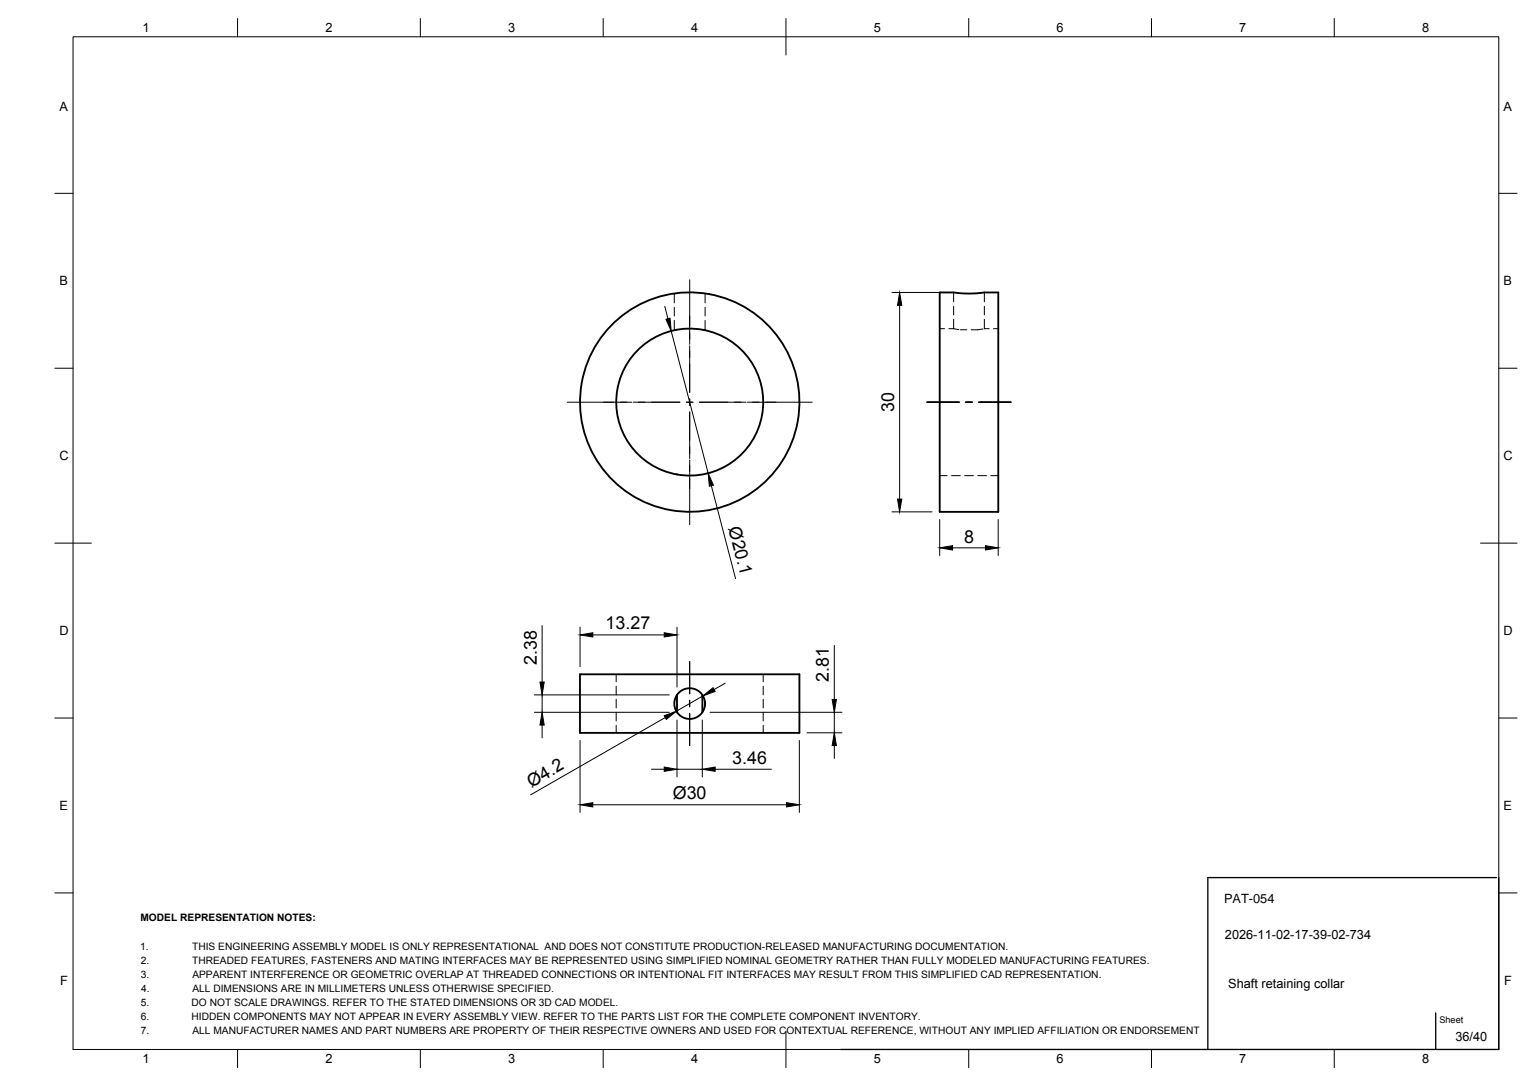
ISO-10303-21;
HEADER;
/* Generated by software containing ST-Developer
 * from STEP Tools, Inc. (www.steptools.com) 
 */

FILE_DESCRIPTION(
/* description */ ('PAT-054'),
/* implementation_level */ '2;1');

FILE_NAME(
/* name */ 'Shaft retaining collar.step',
/* time_stamp */ '2026-10-29T16:38:13-07:00',
/* author */ (''),
/* organization */ (''),
/* preprocessor_version */ 'ST-DEVELOPER v20.2',
/* originating_system */ 'Autodesk Translation Framework v15.17.0.0',
/* authorisation */ '');

FILE_SCHEMA (('AUTOMOTIVE_DESIGN { 1 0 10303 214 3 1 1 }'));
ENDSEC;

DATA;
#10=MECHANICAL_DESIGN_GEOMETRIC_PRESENTATION_REPRESENTATION('',(#950),#33981);
#737=B_SPLINE_CURVE_WITH_KNOTS('',3,(#33386,#33387,#33388,#33389,#33390,
#33391,#33392,#33393),.UNSPECIFIED.,.F.,.F.,(4,2,2,4),(0.756005737987019,
0.793568827564653,0.872922520054208,0.952276212543762),.UNSPECIFIED.);
#738=B_SPLINE_CURVE_WITH_KNOTS('',3,(#33396,#33397,#33398,#33399,#33400,
#33401,#33402,#33403,#33404,#33405,#33406,#33407,#33408,#33409),
 .UNSPECIFIED.,.F.,.F.,(4,2,2,2,2,2,4),(0.121154929624509,0.158718019202145,
0.238071711691699,0.317425404181254,0.396779096670809,0.476132789160363,
0.513695878738001),.UNSPECIFIED.);
#739=B_SPLINE_CURVE_WITH_KNOTS('',3,(#33410,#33411,#33412,#33413,#33414,
#33415,#33416,#33417),.UNSPECIFIED.,.F.,.F.,(4,2,2,4),(0.952276212543762,
1.03162990503332,1.11098359752287,1.14854668710052),.UNSPECIFIED.);
#740=B_SPLINE_CURVE_WITH_KNOTS('',3,(#33421,#33422,#33423,#33424,#33425,
#33426,#33427,#33428,#33429,#33430),.UNSPECIFIED.,.F.,.F.,(4,2,2,2,4),(0.,
0.0792165807733642,0.158433161546728,0.237648697074572,0.316864232602417),
 .UNSPECIFIED.);
#741=B_SPLINE_CURVE_WITH_KNOTS('',3,(#33431,#33432,#33433,#33434,#33435,
#33436,#33437,#33438,#33439,#33440,#33441,#33442,#33443,#33444,#33445,#33446,
#33447,#33448,#33449,#33450,#33451,#33452,#33453,#33454,#33455,#33456),
 .UNSPECIFIED.,.F.,.F.,(4,2,2,2,2,2,2,2,2,2,2,2,4),(0.316864232602417,0.396079768130261,
0.475295303658105,0.554511884431469,0.633728465204833,0.712945045978197,
0.792161626751562,0.871377162279406,0.95059269780725,1.02980823333509,1.10902376886294,
1.1882403496363,1.26745693040967),.UNSPECIFIED.);
#847=SHAPE_REPRESENTATION_RELATIONSHIP('SRR','None',#34225,#891);
#891=ADVANCED_BREP_SHAPE_REPRESENTATION('',(#1005),#33973);
#950=STYLED_ITEM('',(#34517),#1005);
#1005=MANIFOLD_SOLID_BREP('Body1',#13065);
#1210=FACE_BOUND('',#3152,.T.);
#1211=FACE_BOUND('',#3154,.T.);
#1212=FACE_BOUND('',#3156,.T.);
#1213=FACE_BOUND('',#3158,.T.);
#1527=PLANE('',#14711);
#1528=PLANE('',#14715);
#1529=PLANE('',#14722);
#1530=PLANE('',#14723);
#2227=FACE_OUTER_BOUND('',#3148,.T.);
#2228=FACE_OUTER_BOUND('',#3149,.T.);
#2229=FACE_OUTER_BOUND('',#3150,.T.);
#2230=FACE_OUTER_BOUND('',#3151,.T.);
#2231=FACE_OUTER_BOUND('',#3153,.T.);
#2232=FACE_OUTER_BOUND('',#3155,.T.);
#2233=FACE_OUTER_BOUND('',#3157,.T.);
#3148=EDGE_LOOP('',(#11681,#11682));
#3149=EDGE_LOOP('',(#11683,#11684,#11685,#11686,#11687,#11688,#11689,#11690,
#11691));
#3150=EDGE_LOOP('',(#11692,#11693));
#3151=EDGE_LOOP('',(#11694,#11695,#11696,#11697));
#3152=EDGE_LOOP('',(#11698,#11699,#11700,#11701,#11702));
#3153=EDGE_LOOP('',(#11703,#11704,#11705,#11706));
#3154=EDGE_LOOP('',(#11707,#11708));
#3155=EDGE_LOOP('',(#11709));
#3156=EDGE_LOOP('',(#11710));
#3157=EDGE_LOOP('',(#11711));
#3158=EDGE_LOOP('',(#11712));
#4072=LINE('',#33381,#5006);
#4073=LINE('',#33419,#5007);
#4074=LINE('',#33458,#5008);
#4075=LINE('',#33463,#5009);
#4076=LINE('',#33469,#5010);
#5006=VECTOR('',#18031,1.);
#5007=VECTOR('',#18038,0.210000000000001);
#5008=VECTOR('',#18041,1.);
#5009=VECTOR('',#18046,1.005);
#5010=VECTOR('',#18053,1.5);
#5530=CIRCLE('',#14712,0.210000000000001);
#5531=CIRCLE('',#14714,0.210000000000001);
#5532=CIRCLE('',#14717,1.005);
#5533=CIRCLE('',#14718,1.005);
#5534=CIRCLE('',#14720,1.5);
#5535=CIRCLE('',#14721,1.5);
#6646=VERTEX_POINT('',#33379);
#6647=VERTEX_POINT('',#33380);
#6648=VERTEX_POINT('',#33384);
#6649=VERTEX_POINT('',#33385);
#6650=VERTEX_POINT('',#33394);
#6651=VERTEX_POINT('',#33418);
#6652=VERTEX_POINT('',#33420);
#6653=VERTEX_POINT('',#33460);
#6654=VERTEX_POINT('',#33462);
#6655=VERTEX_POINT('',#33466);
#6656=VERTEX_POINT('',#33468);
#8340=EDGE_CURVE('',#6646,#6647,#4072,.T.);
#8341=EDGE_CURVE('',#6646,#6647,#5530,.T.);
#8342=EDGE_CURVE('',#6648,#6649,#737,.T.);
#8343=EDGE_CURVE('',#6650,#6648,#5531,.T.);
#8344=EDGE_CURVE('',#6647,#6650,#738,.T.);
#8345=EDGE_CURVE('',#6649,#6646,#739,.T.);
#8346=EDGE_CURVE('',#6649,#6651,#4073,.T.);
#8347=EDGE_CURVE('',#6652,#6651,#740,.T.);
#8348=EDGE_CURVE('',#6651,#6652,#741,.T.);
#8349=EDGE_CURVE('',#6650,#6648,#4074,.T.);
#8350=EDGE_CURVE('',#6653,#6653,#5532,.T.);
#8351=EDGE_CURVE('',#6653,#6654,#4075,.T.);
#8352=EDGE_CURVE('',#6654,#6654,#5533,.T.);
#8353=EDGE_CURVE('',#6655,#6655,#5534,.T.);
#8354=EDGE_CURVE('',#6655,#6656,#4076,.T.);
#8355=EDGE_CURVE('',#6656,#6656,#5535,.T.);
#11681=ORIENTED_EDGE('',*,*,#8340,.F.);
#11682=ORIENTED_EDGE('',*,*,#8341,.T.);
#11683=ORIENTED_EDGE('',*,*,#8342,.F.);
#11684=ORIENTED_EDGE('',*,*,#8343,.F.);
#11685=ORIENTED_EDGE('',*,*,#8344,.F.);
#11686=ORIENTED_EDGE('',*,*,#8341,.F.);
#11687=ORIENTED_EDGE('',*,*,#8345,.F.);
#11688=ORIENTED_EDGE('',*,*,#8346,.T.);
#11689=ORIENTED_EDGE('',*,*,#8347,.F.);
#11690=ORIENTED_EDGE('',*,*,#8348,.F.);
#11691=ORIENTED_EDGE('',*,*,#8346,.F.);
#11692=ORIENTED_EDGE('',*,*,#8349,.F.);
#11693=ORIENTED_EDGE('',*,*,#8343,.T.);
#11694=ORIENTED_EDGE('',*,*,#8350,.F.);
#11695=ORIENTED_EDGE('',*,*,#8351,.T.);
#11696=ORIENTED_EDGE('',*,*,#8352,.T.);
#11697=ORIENTED_EDGE('',*,*,#8351,.F.);
#11698=ORIENTED_EDGE('',*,*,#8344,.T.);
#11699=ORIENTED_EDGE('',*,*,#8349,.T.);
#11700=ORIENTED_EDGE('',*,*,#8342,.T.);
#11701=ORIENTED_EDGE('',*,*,#8345,.T.);
#11702=ORIENTED_EDGE('',*,*,#8340,.T.);
#11703=ORIENTED_EDGE('',*,*,#8353,.F.);
#11704=ORIENTED_EDGE('',*,*,#8354,.T.);
#11705=ORIENTED_EDGE('',*,*,#8355,.T.);
#11706=ORIENTED_EDGE('',*,*,#8354,.F.);
#11707=ORIENTED_EDGE('',*,*,#8347,.T.);
#11708=ORIENTED_EDGE('',*,*,#8348,.T.);
#11709=ORIENTED_EDGE('',*,*,#8353,.T.);
#11710=ORIENTED_EDGE('',*,*,#8350,.T.);
#11711=ORIENTED_EDGE('',*,*,#8355,.F.);
#11712=ORIENTED_EDGE('',*,*,#8352,.F.);
#12270=CYLINDRICAL_SURFACE('',#14713,0.210000000000001);
#12271=CYLINDRICAL_SURFACE('',#14716,1.005);
#12272=CYLINDRICAL_SURFACE('',#14719,1.5);
#12939=ADVANCED_FACE('',(#2227),#1527,.T.);
#12940=ADVANCED_FACE('',(#2228),#12270,.F.);
#12941=ADVANCED_FACE('',(#2229),#1528,.T.);
#12942=ADVANCED_FACE('',(#2230,#1210),#12271,.F.);
#12943=ADVANCED_FACE('',(#2231,#1211),#12272,.T.);
#12944=ADVANCED_FACE('',(#2232,#1212),#1529,.T.);
#12945=ADVANCED_FACE('',(#2233,#1213),#1530,.F.);
#13065=CLOSED_SHELL('',(#12939,#12940,#12941,#12942,#12943,#12944,#12945));
#14710=AXIS2_PLACEMENT_3D('',#33377,#18027,#18028);
#14711=AXIS2_PLACEMENT_3D('',#33378,#18029,#18030);
#14712=AXIS2_PLACEMENT_3D('',#33382,#18032,#18033);
#14713=AXIS2_PLACEMENT_3D('',#33383,#18034,#18035);
#14714=AXIS2_PLACEMENT_3D('',#33395,#18036,#18037);
#14715=AXIS2_PLACEMENT_3D('',#33457,#18039,#18040);
#14716=AXIS2_PLACEMENT_3D('',#33459,#18042,#18043);
#14717=AXIS2_PLACEMENT_3D('',#33461,#18044,#18045);
#14718=AXIS2_PLACEMENT_3D('',#33464,#18047,#18048);
#14719=AXIS2_PLACEMENT_3D('',#33465,#18049,#18050);
#14720=AXIS2_PLACEMENT_3D('',#33467,#18051,#18052);
#14721=AXIS2_PLACEMENT_3D('',#33470,#18054,#18055);
#14722=AXIS2_PLACEMENT_3D('',#33471,#18056,#18057);
#14723=AXIS2_PLACEMENT_3D('',#33472,#18058,#18059);
#18027=DIRECTION('axis',(0.,0.,1.));
#18028=DIRECTION('refdir',(1.,0.,0.));
#18029=DIRECTION('center_axis',(0.,1.,0.));
#18030=DIRECTION('ref_axis',(1.,0.,0.));
#18031=DIRECTION('',(1.,0.,0.));
#18032=DIRECTION('center_axis',(0.,1.,0.));
#18033=DIRECTION('ref_axis',(1.,0.,0.));
#18034=DIRECTION('center_axis',(0.,1.,0.));
#18035=DIRECTION('ref_axis',(1.,0.,0.));
#18036=DIRECTION('center_axis',(0.,1.,0.));
#18037=DIRECTION('ref_axis',(1.,0.,0.));
#18038=DIRECTION('',(0.,1.,0.));
#18039=DIRECTION('center_axis',(0.,1.,0.));
#18040=DIRECTION('ref_axis',(1.,0.,0.));
#18041=DIRECTION('',(-1.,0.,0.));
#18042=DIRECTION('center_axis',(1.,0.,0.));
#18043=DIRECTION('ref_axis',(0.,0.,-1.));
#18044=DIRECTION('center_axis',(-1.,0.,0.));
#18045=DIRECTION('ref_axis',(0.,0.,-1.));
#18046=DIRECTION('',(-1.,0.,0.));
#18047=DIRECTION('center_axis',(-1.,0.,0.));
#18048=DIRECTION('ref_axis',(0.,0.,-1.));
#18049=DIRECTION('center_axis',(1.,0.,0.));
#18050=DIRECTION('ref_axis',(0.,0.,-1.));
#18051=DIRECTION('center_axis',(1.,0.,0.));
#18052=DIRECTION('ref_axis',(0.,0.,-1.));
#18053=DIRECTION('',(-1.,0.,0.));
#18054=DIRECTION('center_axis',(1.,0.,0.));
#18055=DIRECTION('ref_axis',(0.,0.,-1.));
#18056=DIRECTION('center_axis',(1.,0.,0.));
#18057=DIRECTION('ref_axis',(0.,0.,-1.));
#18058=DIRECTION('center_axis',(1.,0.,0.));
#18059=DIRECTION('ref_axis',(0.,0.,-1.));
#33377=CARTESIAN_POINT('',(0.,0.,0.));
#33378=CARTESIAN_POINT('Origin',(25.8,0.99,4.));
#33379=CARTESIAN_POINT('',(25.6809411910021,0.99,4.17298843892006));
#33380=CARTESIAN_POINT('',(25.9190588089979,0.99,4.17298843892006));
#33381=CARTESIAN_POINT('',(25.4,0.99,4.17298843892006));
#33382=CARTESIAN_POINT('Origin',(25.8,0.99,4.));
#33383=CARTESIAN_POINT('Origin',(25.8,0.99,4.));
#33384=CARTESIAN_POINT('',(25.6809411910021,0.99,3.82701156107994));
#33385=CARTESIAN_POINT('',(25.59,1.005,4.));
#33386=CARTESIAN_POINT('Ctrl Pts',(25.6809411910021,0.989999999999999,3.82701156107994));
#33387=CARTESIAN_POINT('Ctrl Pts',(25.6701985776047,0.99129192197638,3.83440513468868));
#33388=CARTESIAN_POINT('Ctrl Pts',(25.6603122906273,0.992653949439047,3.84270286127439));
#33389=CARTESIAN_POINT('Ctrl Pts',(25.6329072257467,0.996748084390898,3.87010792615492));
#33390=CARTESIAN_POINT('Ctrl Pts',(25.6167579436671,0.999695893276376,3.89366983224072));
#33391=CARTESIAN_POINT('Ctrl Pts',(25.5953022060351,1.00385029472357,3.94538709536759));
#33392=CARTESIAN_POINT('Ctrl Pts',(25.59,1.005,3.97354876917015));
#33393=CARTESIAN_POINT('Ctrl Pts',(25.59,1.005,4.));
#33394=CARTESIAN_POINT('',(25.9190588089979,0.99,3.82701156107994));
#33395=CARTESIAN_POINT('Origin',(25.8,0.99,4.));
#33396=CARTESIAN_POINT('Ctrl Pts',(25.9190588089979,0.99,4.17298843892006));
#33397=CARTESIAN_POINT('Ctrl Pts',(25.9298014223953,0.991291921976381,4.16559486531132));
#33398=CARTESIAN_POINT('Ctrl Pts',(25.9396877093727,0.992653949439047,4.15729713872561));
#33399=CARTESIAN_POINT('Ctrl Pts',(25.9670927742533,0.996748084390898,4.12989207384508));
#33400=CARTESIAN_POINT('Ctrl Pts',(25.9832420563329,0.999695893276376,4.10633016775929));
#33401=CARTESIAN_POINT('Ctrl Pts',(26.0046977939649,1.00385029472357,4.05461290463241));
#33402=CARTESIAN_POINT('Ctrl Pts',(26.01,1.005,4.02645123082985));
#33403=CARTESIAN_POINT('Ctrl Pts',(26.01,1.005,3.97354876917015));
#33404=CARTESIAN_POINT('Ctrl Pts',(26.0046977939649,1.00385029472357,3.94538709536759));
#33405=CARTESIAN_POINT('Ctrl Pts',(25.9832420563329,0.999695893276376,3.89366983224072));
#33406=CARTESIAN_POINT('Ctrl Pts',(25.9670927742533,0.996748084390898,3.87010792615492));
#33407=CARTESIAN_POINT('Ctrl Pts',(25.9396877093727,0.992653949439047,3.84270286127439));
#33408=CARTESIAN_POINT('Ctrl Pts',(25.9298014223953,0.991291921976381,3.83440513468868));
#33409=CARTESIAN_POINT('Ctrl Pts',(25.9190588089979,0.99,3.82701156107994));
#33410=CARTESIAN_POINT('Ctrl Pts',(25.59,1.005,4.));
#33411=CARTESIAN_POINT('Ctrl Pts',(25.59,1.005,4.02645123082985));
#33412=CARTESIAN_POINT('Ctrl Pts',(25.5953022060351,1.00385029472357,4.05461290463241));
#33413=CARTESIAN_POINT('Ctrl Pts',(25.6167579436671,0.999695893276376,4.10633016775929));
#33414=CARTESIAN_POINT('Ctrl Pts',(25.6329072257467,0.996748084390898,4.12989207384508));
#33415=CARTESIAN_POINT('Ctrl Pts',(25.6603122906273,0.992653949439047,4.15729713872561));
#33416=CARTESIAN_POINT('Ctrl Pts',(25.6701985776047,0.991291921976381,4.16559486531132));
#33417=CARTESIAN_POINT('Ctrl Pts',(25.6809411910021,0.99,4.17298843892006));
#33418=CARTESIAN_POINT('',(25.59,1.5,4.));
#33419=CARTESIAN_POINT('',(25.59,0.99,4.));
#33420=CARTESIAN_POINT('',(25.8,1.48522725533839,4.21));
#33421=CARTESIAN_POINT('Ctrl Pts',(25.8,1.48522725533839,4.21));
#33422=CARTESIAN_POINT('Ctrl Pts',(25.7735944730755,1.48522725533839,4.21));
#33423=CARTESIAN_POINT('Ctrl Pts',(25.7454529259093,1.48600415954412,4.2047157372696));
#33424=CARTESIAN_POINT('Ctrl Pts',(25.6937237310949,1.48880073282317,4.18327376303633));
#33425=CARTESIAN_POINT('Ctrl Pts',(25.670133075872,1.49077897157582,4.16711792397039));
#33426=CARTESIAN_POINT('Ctrl Pts',(25.632882321789,1.49448481141327,4.12986716988737));
#33427=CARTESIAN_POINT('Ctrl Pts',(25.6167262899986,1.49645455657129,4.10627640830577));
#33428=CARTESIAN_POINT('Ctrl Pts',(25.5952841751738,1.49923165515646,4.0545468514059));
#33429=CARTESIAN_POINT('Ctrl Pts',(25.59,1.5,4.02640517850928));
#33430=CARTESIAN_POINT('Ctrl Pts',(25.59,1.5,4.));
#33431=CARTESIAN_POINT('Ctrl Pts',(25.59,1.5,4.));
#33432=CARTESIAN_POINT('Ctrl Pts',(25.59,1.5,3.97359482149072));
#33433=CARTESIAN_POINT('Ctrl Pts',(25.5952841751738,1.49923165515646,3.9454531485941));
#33434=CARTESIAN_POINT('Ctrl Pts',(25.6167262899986,1.49645455657129,3.89372359169423));
#33435=CARTESIAN_POINT('Ctrl Pts',(25.632882321789,1.49448481141327,3.87013283011263));
#33436=CARTESIAN_POINT('Ctrl Pts',(25.670133075872,1.49077897157582,3.83288207602961));
#33437=CARTESIAN_POINT('Ctrl Pts',(25.6937237310949,1.48880073282317,3.81672623696366));
#33438=CARTESIAN_POINT('Ctrl Pts',(25.7454529259093,1.48600415954412,3.7952842627304));
#33439=CARTESIAN_POINT('Ctrl Pts',(25.7735944730755,1.48522725533839,3.79));
#33440=CARTESIAN_POINT('Ctrl Pts',(25.8264055269245,1.48522725533839,3.79));
#33441=CARTESIAN_POINT('Ctrl Pts',(25.8545470740907,1.48600415954412,3.7952842627304));
#33442=CARTESIAN_POINT('Ctrl Pts',(25.9062762689051,1.48880073282317,3.81672623696367));
#33443=CARTESIAN_POINT('Ctrl Pts',(25.929866924128,1.49077897157582,3.83288207602961));
#33444=CARTESIAN_POINT('Ctrl Pts',(25.967117678211,1.49448481141327,3.87013283011263));
#33445=CARTESIAN_POINT('Ctrl Pts',(25.9832737100014,1.49645455657129,3.89372359169423));
#33446=CARTESIAN_POINT('Ctrl Pts',(26.0047158248262,1.49923165515646,3.9454531485941));
#33447=CARTESIAN_POINT('Ctrl Pts',(26.01,1.5,3.97359482149072));
#33448=CARTESIAN_POINT('Ctrl Pts',(26.01,1.5,4.02640517850928));
#33449=CARTESIAN_POINT('Ctrl Pts',(26.0047158248262,1.49923165515646,4.0545468514059));
#33450=CARTESIAN_POINT('Ctrl Pts',(25.9832737100014,1.49645455657129,4.10627640830577));
#33451=CARTESIAN_POINT('Ctrl Pts',(25.967117678211,1.49448481141327,4.12986716988737));
#33452=CARTESIAN_POINT('Ctrl Pts',(25.929866924128,1.49077897157582,4.16711792397039));
#33453=CARTESIAN_POINT('Ctrl Pts',(25.9062762689051,1.48880073282317,4.18327376303633));
#33454=CARTESIAN_POINT('Ctrl Pts',(25.8545470740907,1.48600415954412,4.20471573726959));
#33455=CARTESIAN_POINT('Ctrl Pts',(25.8264055269245,1.48522725533839,4.21));
#33456=CARTESIAN_POINT('Ctrl Pts',(25.8,1.48522725533839,4.21));
#33457=CARTESIAN_POINT('Origin',(25.8,0.99,4.));
#33458=CARTESIAN_POINT('',(25.4,0.99,3.82701156107994));
#33459=CARTESIAN_POINT('Origin',(25.4,0.,4.));
#33460=CARTESIAN_POINT('',(26.2,-1.23077003314309E-16,5.005));
#33461=CARTESIAN_POINT('Origin',(26.2,0.,4.));
#33462=CARTESIAN_POINT('',(25.4,-1.23077003314309E-16,5.005));
#33463=CARTESIAN_POINT('',(25.4,-1.23077003314309E-16,5.005));
#33464=CARTESIAN_POINT('Origin',(25.4,0.,4.));
#33465=CARTESIAN_POINT('Origin',(25.4,0.,4.));
#33466=CARTESIAN_POINT('',(26.2,-1.83697019872103E-16,5.5));
#33467=CARTESIAN_POINT('Origin',(26.2,0.,4.));
#33468=CARTESIAN_POINT('',(25.4,-1.83697019872103E-16,5.5));
#33469=CARTESIAN_POINT('',(25.4,-1.83697019872103E-16,5.5));
#33470=CARTESIAN_POINT('Origin',(25.4,0.,4.));
#33471=CARTESIAN_POINT('Origin',(26.2,0.,4.));
#33472=CARTESIAN_POINT('Origin',(25.4,0.,4.));
#33921=UNCERTAINTY_MEASURE_WITH_UNIT(LENGTH_MEASURE(0.001),#33982,
'DISTANCE_ACCURACY_VALUE',
'Maximum model space distance between geometric entities at asserted c
onnectivities');
#33929=UNCERTAINTY_MEASURE_WITH_UNIT(LENGTH_MEASURE(0.001),#33982,
'DISTANCE_ACCURACY_VALUE',
'Maximum model space distance between geometric entities at asserted c
onnectivities');
#33973=(
GEOMETRIC_REPRESENTATION_CONTEXT(3)
GLOBAL_UNCERTAINTY_ASSIGNED_CONTEXT((#33921))
GLOBAL_UNIT_ASSIGNED_CONTEXT((#33982,#33984,#33985))
REPRESENTATION_CONTEXT('','3D')
);
#33981=(
GEOMETRIC_REPRESENTATION_CONTEXT(3)
GLOBAL_UNCERTAINTY_ASSIGNED_CONTEXT((#33929))
GLOBAL_UNIT_ASSIGNED_CONTEXT((#33982,#33984,#33985))
REPRESENTATION_CONTEXT('','3D')
);
#33982=(
LENGTH_UNIT()
NAMED_UNIT(*)
SI_UNIT(.CENTI.,.METRE.)
);
#33984=(
NAMED_UNIT(*)
PLANE_ANGLE_UNIT()
SI_UNIT($,.RADIAN.)
);
#33985=(
NAMED_UNIT(*)
SI_UNIT($,.STERADIAN.)
SOLID_ANGLE_UNIT()
);
#34029=SHAPE_DEFINITION_REPRESENTATION(#34113,#34225);
#34113=PRODUCT_DEFINITION_SHAPE('',$,#34277);
#34225=SHAPE_REPRESENTATION('',(#14710),#33973);
#34233=PRODUCT_DEFINITION_CONTEXT('part definition',#34388,'design');
#34277=PRODUCT_DEFINITION('Shaft retaining collar',
'Shaft retaining collar',#34328,#34233);
#34328=PRODUCT_DEFINITION_FORMATION('',$,#34433);
#34388=APPLICATION_CONTEXT(
'Core Data for Automotive Mechanical Design Process');
#34389=PRODUCT_CONTEXT('part definition',#34388,'mechanical');
#34433=PRODUCT('Shaft retaining collar','Shaft retaining collar',
'Shaft retaining collar',(#34389));
#34511=COLOUR_RGB('Grey',0.48,0.52,0.57);
#34512=FILL_AREA_STYLE_COLOUR('',#34511);
#34513=FILL_AREA_STYLE('',(#34512));
#34514=SURFACE_STYLE_FILL_AREA(#34513);
#34515=SURFACE_SIDE_STYLE('',(#34514));
#34516=SURFACE_STYLE_USAGE(.BOTH.,#34515);
#34517=PRESENTATION_STYLE_ASSIGNMENT((#34516));
ENDSEC;
END-ISO-10303-21;
